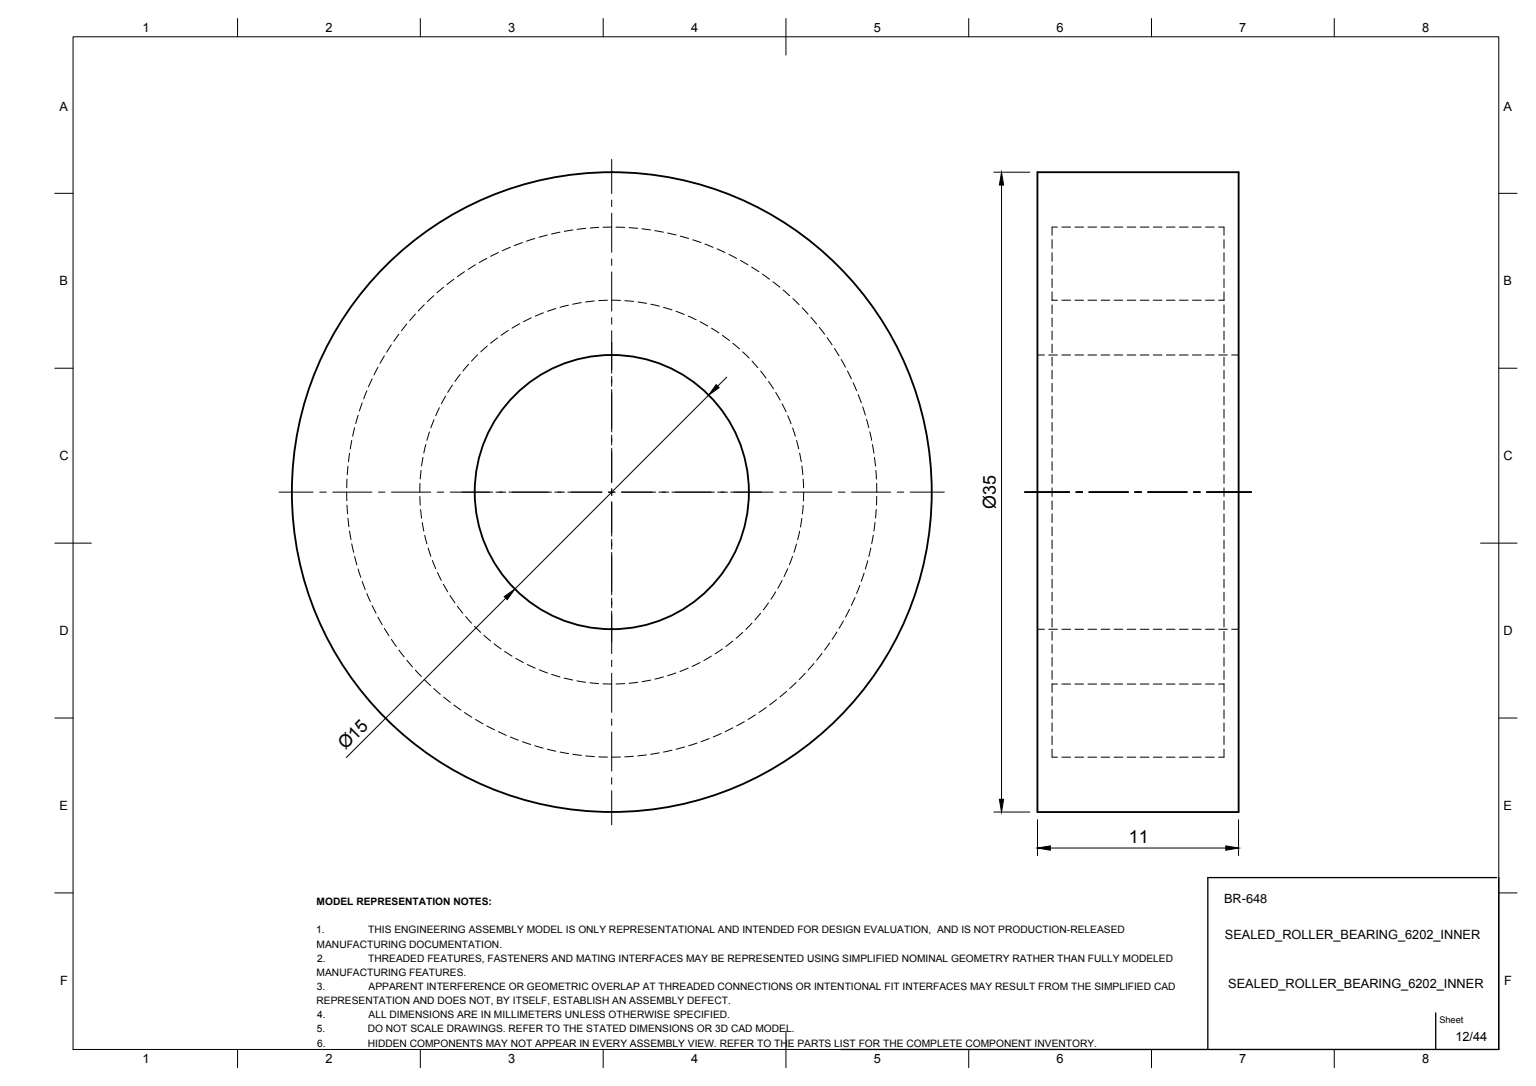
ISO-10303-21;
HEADER;
FILE_DESCRIPTION((''),'2;1');
FILE_NAME('SEALED_ROLLER_BEARING_6202_INNER.step','2026-10-01T22:05:39-07:00',(''),(''),'','','');
FILE_SCHEMA (('AUTOMOTIVE_DESIGN { 1 0 10303 214 3 1 1 }'));
ENDSEC;
DATA;
#10=MECHANICAL_DESIGN_GEOMETRIC_PRESENTATION_REPRESENTATION('',(#612),#24628);
#486=ORIENTED_CLOSED_SHELL('',*,#13122,.F.) ;
#519=BREP_WITH_VOIDS('SEALED_ROLLER_BEARING_6202_INNER',#13123,(#486)) ;
#528=SHAPE_REPRESENTATION_RELATIONSHIP('SRR','None',#24800,#570) ;
#570=ADVANCED_BREP_SHAPE_REPRESENTATION('',(#519),#24590) ;
#612=STYLED_ITEM('',(#25034),#519) ;
#843=FACE_BOUND('',#4057,.T.) ;
#844=FACE_BOUND('',#4059,.T.) ;
#845=FACE_BOUND('',#4063,.T.) ;
#846=FACE_BOUND('',#4066,.T.) ;
#1146=LINE('',#20650,#1982) ;
#1147=LINE('',#20652,#1983) ;
#1148=LINE('',#20661,#1984) ;
#1149=LINE('',#20666,#1985) ;
#1982=VECTOR('',#16403,1.05) ;
#1983=VECTOR('',#16406,1.45) ;
#1984=VECTOR('',#16417,1.75) ;
#1985=VECTOR('',#16424,0.75) ;
#2782=CYLINDRICAL_SURFACE('',#14085,1.05) ;
#2783=CYLINDRICAL_SURFACE('',#14086,1.45) ;
#2784=CYLINDRICAL_SURFACE('',#14090,1.75) ;
#2785=CYLINDRICAL_SURFACE('',#14094,0.75) ;
#3132=FACE_OUTER_BOUND('',#4056,.T.) ;
#3133=FACE_OUTER_BOUND('',#4058,.T.) ;
#3134=FACE_OUTER_BOUND('',#4060,.T.) ;
#3135=FACE_OUTER_BOUND('',#4061,.T.) ;
#3136=FACE_OUTER_BOUND('',#4062,.T.) ;
#3137=FACE_OUTER_BOUND('',#4064,.T.) ;
#3138=FACE_OUTER_BOUND('',#4065,.T.) ;
#3139=FACE_OUTER_BOUND('',#4067,.T.) ;
#4056=EDGE_LOOP('',(#9261)) ;
#4057=EDGE_LOOP('',(#9262)) ;
#4058=EDGE_LOOP('',(#9263)) ;
#4059=EDGE_LOOP('',(#9264)) ;
#4060=EDGE_LOOP('',(#9265,#9266,#9267,#9268)) ;
#4061=EDGE_LOOP('',(#9269,#9270,#9271,#9272)) ;
#4062=EDGE_LOOP('',(#9273)) ;
#4063=EDGE_LOOP('',(#9274)) ;
#4064=EDGE_LOOP('',(#9275,#9276,#9277,#9278)) ;
#4065=EDGE_LOOP('',(#9279)) ;
#4066=EDGE_LOOP('',(#9280)) ;
#4067=EDGE_LOOP('',(#9281,#9282,#9283,#9284)) ;
#4988=CIRCLE('',#14080,1.45) ;
#4989=CIRCLE('',#14081,1.05) ;
#4990=CIRCLE('',#14083,1.45) ;
#4991=CIRCLE('',#14084,1.05) ;
#4992=CIRCLE('',#14088,1.75) ;
#4993=CIRCLE('',#14089,0.75) ;
#4994=CIRCLE('',#14091,1.75) ;
#4995=CIRCLE('',#14093,0.75) ;
#5795=VERTEX_POINT('',#20640) ;
#5796=VERTEX_POINT('',#20642) ;
#5797=VERTEX_POINT('',#20645) ;
#5798=VERTEX_POINT('',#20647) ;
#5799=VERTEX_POINT('',#20654) ;
#5800=VERTEX_POINT('',#20656) ;
#5801=VERTEX_POINT('',#20659) ;
#5802=VERTEX_POINT('',#20663) ;
#7120=EDGE_CURVE('',#5795,#5795,#4988,.T.) ;
#7121=EDGE_CURVE('',#5796,#5796,#4989,.T.) ;
#7122=EDGE_CURVE('',#5797,#5797,#4990,.T.) ;
#7123=EDGE_CURVE('',#5798,#5798,#4991,.T.) ;
#7124=EDGE_CURVE('',#5796,#5798,#1146,.T.) ;
#7125=EDGE_CURVE('',#5797,#5795,#1147,.T.) ;
#7126=EDGE_CURVE('',#5799,#5799,#4992,.T.) ;
#7127=EDGE_CURVE('',#5800,#5800,#4993,.T.) ;
#7128=EDGE_CURVE('',#5801,#5801,#4994,.T.) ;
#7129=EDGE_CURVE('',#5801,#5799,#1148,.T.) ;
#7130=EDGE_CURVE('',#5802,#5802,#4995,.T.) ;
#7131=EDGE_CURVE('',#5800,#5802,#1149,.T.) ;
#9261=ORIENTED_EDGE('',*,*,#7120,.F.) ;
#9262=ORIENTED_EDGE('',*,*,#7121,.F.) ;
#9263=ORIENTED_EDGE('',*,*,#7122,.F.) ;
#9264=ORIENTED_EDGE('',*,*,#7123,.F.) ;
#9265=ORIENTED_EDGE('',*,*,#7121,.T.) ;
#9266=ORIENTED_EDGE('',*,*,#7124,.T.) ;
#9267=ORIENTED_EDGE('',*,*,#7123,.T.) ;
#9268=ORIENTED_EDGE('',*,*,#7124,.F.) ;
#9269=ORIENTED_EDGE('',*,*,#7122,.T.) ;
#9270=ORIENTED_EDGE('',*,*,#7125,.T.) ;
#9271=ORIENTED_EDGE('',*,*,#7120,.T.) ;
#9272=ORIENTED_EDGE('',*,*,#7125,.F.) ;
#9273=ORIENTED_EDGE('',*,*,#7126,.T.) ;
#9274=ORIENTED_EDGE('',*,*,#7127,.T.) ;
#9275=ORIENTED_EDGE('',*,*,#7128,.F.) ;
#9276=ORIENTED_EDGE('',*,*,#7129,.T.) ;
#9277=ORIENTED_EDGE('',*,*,#7126,.F.) ;
#9278=ORIENTED_EDGE('',*,*,#7129,.F.) ;
#9279=ORIENTED_EDGE('',*,*,#7128,.T.) ;
#9280=ORIENTED_EDGE('',*,*,#7130,.T.) ;
#9281=ORIENTED_EDGE('',*,*,#7127,.F.) ;
#9282=ORIENTED_EDGE('',*,*,#7131,.T.) ;
#9283=ORIENTED_EDGE('',*,*,#7130,.F.) ;
#9284=ORIENTED_EDGE('',*,*,#7131,.F.) ;
#12066=PLANE('',#14079) ;
#12067=PLANE('',#14082) ;
#12068=PLANE('',#14087) ;
#12069=PLANE('',#14092) ;
#12527=ADVANCED_FACE('',(#3132,#843),#12066,.T.) ;
#12528=ADVANCED_FACE('',(#3133,#844),#12067,.T.) ;
#12529=ADVANCED_FACE('',(#3134),#2782,.T.) ;
#12530=ADVANCED_FACE('',(#3135),#2783,.F.) ;
#12531=ADVANCED_FACE('',(#3136,#845),#12068,.T.) ;
#12532=ADVANCED_FACE('',(#3137),#2784,.T.) ;
#12533=ADVANCED_FACE('',(#3138,#846),#12069,.T.) ;
#12534=ADVANCED_FACE('',(#3139),#2785,.F.) ;
#13122=CLOSED_SHELL('',(#12527,#12528,#12529,#12530)) ;
#13123=CLOSED_SHELL('',(#12531,#12532,#12533,#12534)) ;
#14078=AXIS2_PLACEMENT_3D('',#20638,#16387,#16388) ;
#14079=AXIS2_PLACEMENT_3D('',#20639,#16389,#16390) ;
#14080=AXIS2_PLACEMENT_3D('',#20641,#16391,#16392) ;
#14081=AXIS2_PLACEMENT_3D('',#20643,#16393,#16394) ;
#14082=AXIS2_PLACEMENT_3D('',#20644,#16395,#16396) ;
#14083=AXIS2_PLACEMENT_3D('',#20646,#16397,#16398) ;
#14084=AXIS2_PLACEMENT_3D('',#20648,#16399,#16400) ;
#14085=AXIS2_PLACEMENT_3D('',#20649,#16401,#16402) ;
#14086=AXIS2_PLACEMENT_3D('',#20651,#16404,#16405) ;
#14087=AXIS2_PLACEMENT_3D('',#20653,#16407,#16408) ;
#14088=AXIS2_PLACEMENT_3D('',#20655,#16409,#16410) ;
#14089=AXIS2_PLACEMENT_3D('',#20657,#16411,#16412) ;
#14090=AXIS2_PLACEMENT_3D('',#20658,#16413,#16414) ;
#14091=AXIS2_PLACEMENT_3D('',#20660,#16415,#16416) ;
#14092=AXIS2_PLACEMENT_3D('',#20662,#16418,#16419) ;
#14093=AXIS2_PLACEMENT_3D('',#20664,#16420,#16421) ;
#14094=AXIS2_PLACEMENT_3D('',#20665,#16422,#16423) ;
#16387=DIRECTION('axis',(0.,0.,1.)) ;
#16388=DIRECTION('refdir',(1.,0.,0.)) ;
#16389=DIRECTION('center_axis',(0.,-1.,0.)) ;
#16390=DIRECTION('ref_axis',(-1.,0.,0.)) ;
#16391=DIRECTION('center_axis',(0.,1.,0.)) ;
#16392=DIRECTION('ref_axis',(1.,0.,0.)) ;
#16393=DIRECTION('center_axis',(0.,-1.,0.)) ;
#16394=DIRECTION('ref_axis',(1.,0.,0.)) ;
#16395=DIRECTION('center_axis',(0.,1.,0.)) ;
#16396=DIRECTION('ref_axis',(1.,0.,0.)) ;
#16397=DIRECTION('center_axis',(0.,-1.,0.)) ;
#16398=DIRECTION('ref_axis',(1.,0.,0.)) ;
#16399=DIRECTION('center_axis',(0.,1.,0.)) ;
#16400=DIRECTION('ref_axis',(1.,0.,0.)) ;
#16401=DIRECTION('center_axis',(0.,1.,0.)) ;
#16402=DIRECTION('ref_axis',(1.,0.,0.)) ;
#16403=DIRECTION('',(0.,-1.,0.)) ;
#16404=DIRECTION('center_axis',(0.,1.,0.)) ;
#16405=DIRECTION('ref_axis',(1.,0.,0.)) ;
#16406=DIRECTION('',(0.,1.,0.)) ;
#16407=DIRECTION('center_axis',(0.,-1.,0.)) ;
#16408=DIRECTION('ref_axis',(-1.,0.,0.)) ;
#16409=DIRECTION('center_axis',(0.,-1.,0.)) ;
#16410=DIRECTION('ref_axis',(1.,0.,0.)) ;
#16411=DIRECTION('center_axis',(0.,1.,0.)) ;
#16412=DIRECTION('ref_axis',(1.,0.,0.)) ;
#16413=DIRECTION('center_axis',(0.,1.,0.)) ;
#16414=DIRECTION('ref_axis',(1.,0.,0.)) ;
#16415=DIRECTION('center_axis',(0.,1.,0.)) ;
#16416=DIRECTION('ref_axis',(1.,0.,0.)) ;
#16417=DIRECTION('',(0.,-1.,0.)) ;
#16418=DIRECTION('center_axis',(0.,1.,0.)) ;
#16419=DIRECTION('ref_axis',(1.,0.,0.)) ;
#16420=DIRECTION('center_axis',(0.,-1.,0.)) ;
#16421=DIRECTION('ref_axis',(1.,0.,0.)) ;
#16422=DIRECTION('center_axis',(0.,1.,0.)) ;
#16423=DIRECTION('ref_axis',(1.,0.,0.)) ;
#16424=DIRECTION('',(0.,1.,0.)) ;
#20638=CARTESIAN_POINT('',(0.,0.,0.)) ;
#20639=CARTESIAN_POINT('Origin',(0.,-2.58,0.)) ;
#20640=CARTESIAN_POINT('',(-1.45,-2.58,1.77573785876366E-16)) ;
#20641=CARTESIAN_POINT('Origin',(0.,-2.58,0.)) ;
#20642=CARTESIAN_POINT('',(-1.05,-2.58,-1.28587913910472E-16)) ;
#20643=CARTESIAN_POINT('Origin',(0.,-2.58,0.)) ;
#20644=CARTESIAN_POINT('Origin',(0.,-3.52,0.)) ;
#20645=CARTESIAN_POINT('',(-1.45,-3.52,-1.77573785876366E-16)) ;
#20646=CARTESIAN_POINT('Origin',(0.,-3.52,0.)) ;
#20647=CARTESIAN_POINT('',(-1.05,-3.52,1.28587913910472E-16)) ;
#20648=CARTESIAN_POINT('Origin',(0.,-3.52,0.)) ;
#20649=CARTESIAN_POINT('Origin',(0.,-3.05,0.)) ;
#20650=CARTESIAN_POINT('',(-1.05,-3.05,1.28587913910472E-16)) ;
#20651=CARTESIAN_POINT('Origin',(0.,-3.05,0.)) ;
#20652=CARTESIAN_POINT('',(-1.45,-3.05,1.77573785876366E-16)) ;
#20653=CARTESIAN_POINT('Origin',(0.,-3.6,0.)) ;
#20654=CARTESIAN_POINT('',(-1.75,-3.6,2.14313189850787E-16)) ;
#20655=CARTESIAN_POINT('Origin',(0.,-3.6,0.)) ;
#20656=CARTESIAN_POINT('',(-0.75,-3.6,9.18485099360515E-17)) ;
#20657=CARTESIAN_POINT('Origin',(0.,-3.6,0.)) ;
#20658=CARTESIAN_POINT('Origin',(0.,-3.05,0.)) ;
#20659=CARTESIAN_POINT('',(-1.75,-2.5,2.14313189850787E-16)) ;
#20660=CARTESIAN_POINT('Origin',(0.,-2.5,0.)) ;
#20661=CARTESIAN_POINT('',(-1.75,-3.05,2.14313189850787E-16)) ;
#20662=CARTESIAN_POINT('Origin',(0.,-2.5,0.)) ;
#20663=CARTESIAN_POINT('',(-0.75,-2.5,-9.18485099360515E-17)) ;
#20664=CARTESIAN_POINT('Origin',(0.,-2.5,0.)) ;
#20665=CARTESIAN_POINT('Origin',(0.,-3.05,0.)) ;
#20666=CARTESIAN_POINT('',(-0.75,-3.05,9.18485099360515E-17)) ;
#24542=UNCERTAINTY_MEASURE_WITH_UNIT(LENGTH_MEASURE(0.001),#24629,
'DISTANCE_ACCURACY_VALUE',
'Maximum model space distance between geometric entities at asserted c
onnectivities') ;
#24580=UNCERTAINTY_MEASURE_WITH_UNIT(LENGTH_MEASURE(0.001),#24629,
'DISTANCE_ACCURACY_VALUE',
'Maximum model space distance between geometric entities at asserted c
onnectivities') ;
#24590=(
GEOMETRIC_REPRESENTATION_CONTEXT(3)
GLOBAL_UNCERTAINTY_ASSIGNED_CONTEXT((#24542))
GLOBAL_UNIT_ASSIGNED_CONTEXT((#24629,#24631,#24632))
REPRESENTATION_CONTEXT('','3D')
) ;
#24628=(
GEOMETRIC_REPRESENTATION_CONTEXT(3)
GLOBAL_UNCERTAINTY_ASSIGNED_CONTEXT((#24580))
GLOBAL_UNIT_ASSIGNED_CONTEXT((#24629,#24631,#24632))
REPRESENTATION_CONTEXT('','3D')
) ;
#24629=(
LENGTH_UNIT()
NAMED_UNIT(*)
SI_UNIT(.CENTI.,.METRE.)
) ;
#24631=(
NAMED_UNIT(*)
PLANE_ANGLE_UNIT()
SI_UNIT($,.RADIAN.)
) ;
#24632=(
NAMED_UNIT(*)
SI_UNIT($,.STERADIAN.)
SOLID_ANGLE_UNIT()
) ;
#24642=SHAPE_DEFINITION_REPRESENTATION(#24689,#24800) ;
#24689=PRODUCT_DEFINITION_SHAPE('',$,#24848) ;
#24800=SHAPE_REPRESENTATION('',(#14078),#24590) ;
#24838=PRODUCT_DEFINITION_CONTEXT('part definition',#24981,'design') ;
#24848=PRODUCT_DEFINITION('SEALED_ROLLER_BEARING_6202_INNER',
'SEALED_ROLLER_BEARING_6202_INNER',#24895,#24838) ;
#24895=PRODUCT_DEFINITION_FORMATION('',$,#24992) ;
#24981=APPLICATION_CONTEXT(
'Core Data for Automotive Mechanical Design Process') ;
#24982=PRODUCT_CONTEXT('part definition',#24981,'mechanical') ;
#24992=PRODUCT('SEALED_ROLLER_BEARING_6202_INNER',
'SEALED_ROLLER_BEARING_6202_INNER',$,(#24982)) ;
#25034=PRESENTATION_STYLE_ASSIGNMENT((#25044)) ;
#25044=SURFACE_STYLE_USAGE(.BOTH.,#25054) ;
#25054=SURFACE_SIDE_STYLE('',(#25064)) ;
#25064=SURFACE_STYLE_FILL_AREA(#25074) ;
#25074=FILL_AREA_STYLE('Stainless Steel - Satin',(#25084)) ;
#25084=FILL_AREA_STYLE_COLOUR('Stainless Steel - Satin',#25094) ;
#25094=COLOUR_RGB('Stainless Steel - Satin', 0.31764706, 0.68627451, 0.89019608) ;
ENDSEC;
END-ISO-10303-21;
